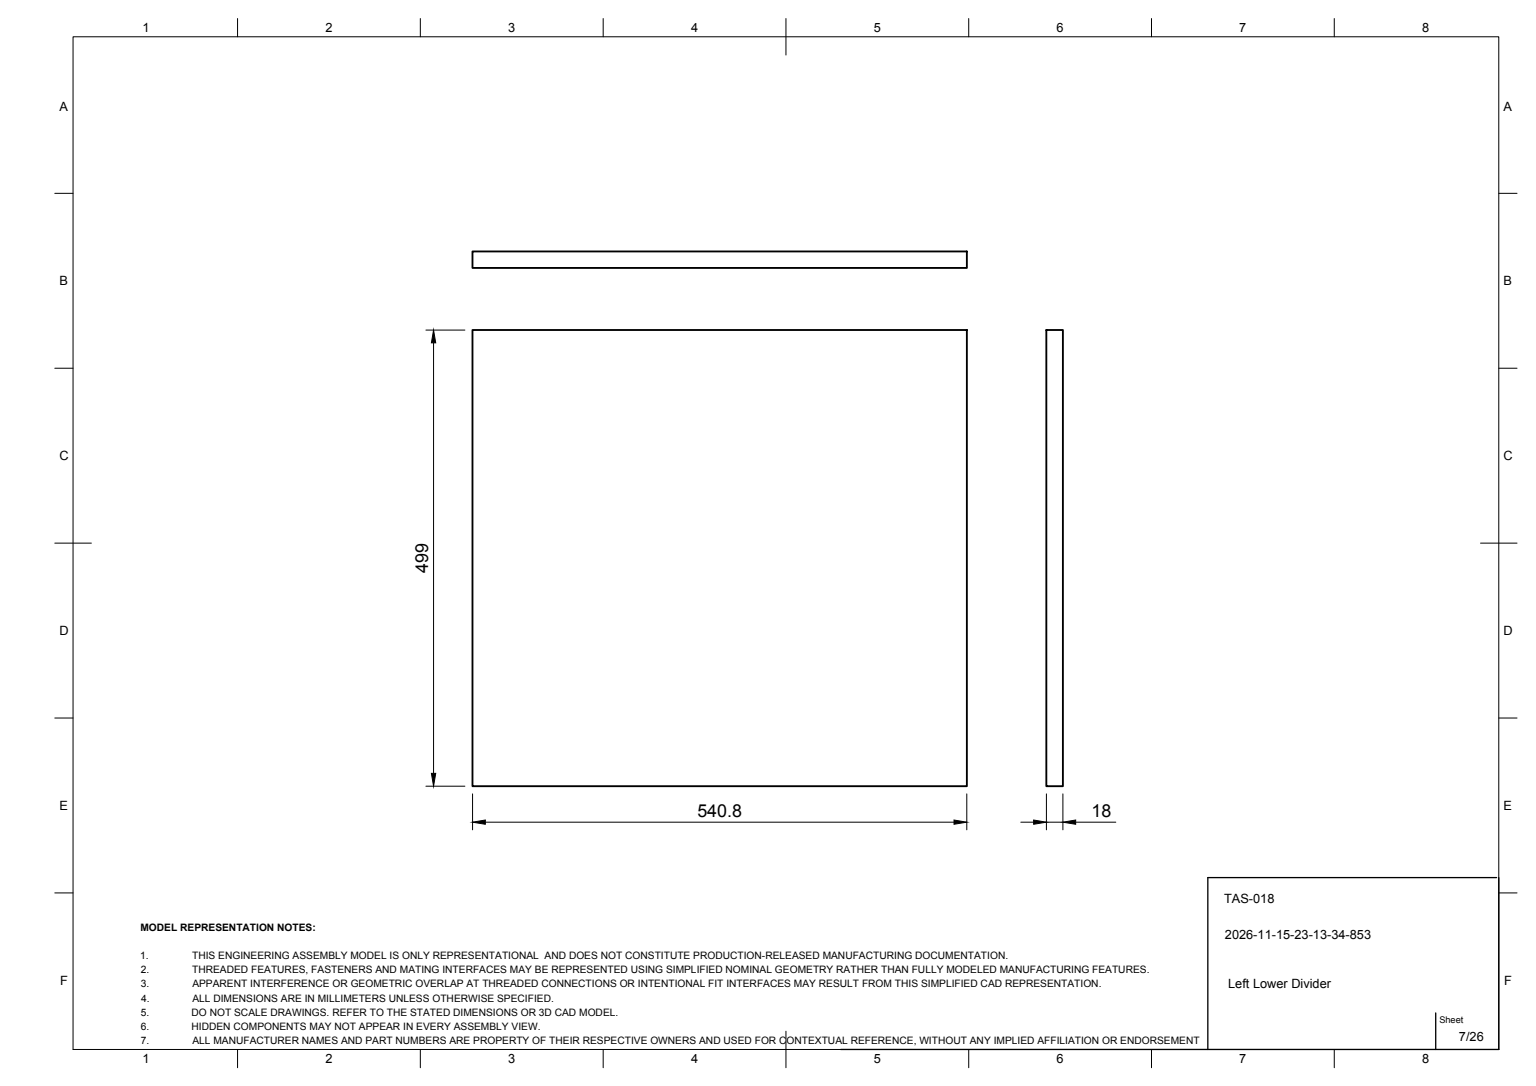
ISO-10303-21;
HEADER;
/* Generated by software containing ST-Developer
 * from STEP Tools, Inc. (www.steptools.com) 
 */

FILE_DESCRIPTION(
/* description */ (''),
/* implementation_level */ '2;1');

FILE_NAME(
/* name */ 'Left Lower Divider.step',
/* time_stamp */ '2026-11-15T15:17:57-08:00',
/* author */ (''),
/* organization */ (''),
/* preprocessor_version */ 'ST-DEVELOPER v20.2',
/* originating_system */ 'Autodesk Translation Framework v15.17.0.0',
/* authorisation */ '');

FILE_SCHEMA (('AUTOMOTIVE_DESIGN { 1 0 10303 214 3 1 1 }'));
ENDSEC;

DATA;
#10=MECHANICAL_DESIGN_GEOMETRIC_PRESENTATION_REPRESENTATION('',(#182),#3723);
#134=SHAPE_REPRESENTATION_RELATIONSHIP('SRR','None',#3815,#158);
#158=ADVANCED_BREP_SHAPE_REPRESENTATION('',(#206),#3704);
#182=STYLED_ITEM('',(#3946),#206);
#206=MANIFOLD_SOLID_BREP('Body1',#2030);
#252=FACE_OUTER_BOUND('',#378,.T.);
#253=FACE_OUTER_BOUND('',#379,.T.);
#254=FACE_OUTER_BOUND('',#380,.T.);
#255=FACE_OUTER_BOUND('',#381,.T.);
#256=FACE_OUTER_BOUND('',#382,.T.);
#257=FACE_OUTER_BOUND('',#383,.T.);
#378=EDGE_LOOP('',(#1413,#1414,#1415,#1416));
#379=EDGE_LOOP('',(#1417,#1418,#1419,#1420));
#380=EDGE_LOOP('',(#1421,#1422,#1423,#1424));
#381=EDGE_LOOP('',(#1425,#1426,#1427,#1428));
#382=EDGE_LOOP('',(#1429,#1430,#1431,#1432));
#383=EDGE_LOOP('',(#1433,#1434,#1435,#1436));
#526=LINE('',#3227,#748);
#527=LINE('',#3229,#749);
#528=LINE('',#3231,#750);
#529=LINE('',#3232,#751);
#530=LINE('',#3235,#752);
#531=LINE('',#3237,#753);
#532=LINE('',#3238,#754);
#533=LINE('',#3241,#755);
#534=LINE('',#3243,#756);
#535=LINE('',#3244,#757);
#536=LINE('',#3246,#758);
#537=LINE('',#3247,#759);
#748=VECTOR('',#2630,21.2913385826772);
#749=VECTOR('',#2631,19.6456692913386);
#750=VECTOR('',#2632,21.2913385826772);
#751=VECTOR('',#2633,19.6456692913386);
#752=VECTOR('',#2636,0.708661417322832);
#753=VECTOR('',#2637,0.708661417322832);
#754=VECTOR('',#2638,21.2913385826772);
#755=VECTOR('',#2641,19.6456692913386);
#756=VECTOR('',#2642,19.6456692913386);
#757=VECTOR('',#2643,21.2913385826772);
#758=VECTOR('',#2646,0.708661417322832);
#759=VECTOR('',#2647,0.708661417322832);
#955=VERTEX_POINT('',#3225);
#956=VERTEX_POINT('',#3226);
#957=VERTEX_POINT('',#3228);
#958=VERTEX_POINT('',#3230);
#959=VERTEX_POINT('',#3234);
#960=VERTEX_POINT('',#3236);
#961=VERTEX_POINT('',#3240);
#962=VERTEX_POINT('',#3242);
#1128=EDGE_CURVE('',#955,#956,#526,.T.);
#1129=EDGE_CURVE('',#955,#957,#527,.T.);
#1130=EDGE_CURVE('',#957,#958,#528,.T.);
#1131=EDGE_CURVE('',#956,#958,#529,.T.);
#1132=EDGE_CURVE('',#955,#959,#530,.T.);
#1133=EDGE_CURVE('',#956,#960,#531,.T.);
#1134=EDGE_CURVE('',#959,#960,#532,.T.);
#1135=EDGE_CURVE('',#959,#961,#533,.T.);
#1136=EDGE_CURVE('',#960,#962,#534,.T.);
#1137=EDGE_CURVE('',#961,#962,#535,.T.);
#1138=EDGE_CURVE('',#961,#957,#536,.T.);
#1139=EDGE_CURVE('',#962,#958,#537,.T.);
#1413=ORIENTED_EDGE('',*,*,#1128,.F.);
#1414=ORIENTED_EDGE('',*,*,#1129,.T.);
#1415=ORIENTED_EDGE('',*,*,#1130,.T.);
#1416=ORIENTED_EDGE('',*,*,#1131,.F.);
#1417=ORIENTED_EDGE('',*,*,#1132,.F.);
#1418=ORIENTED_EDGE('',*,*,#1128,.T.);
#1419=ORIENTED_EDGE('',*,*,#1133,.T.);
#1420=ORIENTED_EDGE('',*,*,#1134,.F.);
#1421=ORIENTED_EDGE('',*,*,#1135,.F.);
#1422=ORIENTED_EDGE('',*,*,#1134,.T.);
#1423=ORIENTED_EDGE('',*,*,#1136,.T.);
#1424=ORIENTED_EDGE('',*,*,#1137,.F.);
#1425=ORIENTED_EDGE('',*,*,#1138,.F.);
#1426=ORIENTED_EDGE('',*,*,#1137,.T.);
#1427=ORIENTED_EDGE('',*,*,#1139,.T.);
#1428=ORIENTED_EDGE('',*,*,#1130,.F.);
#1429=ORIENTED_EDGE('',*,*,#1131,.T.);
#1430=ORIENTED_EDGE('',*,*,#1139,.F.);
#1431=ORIENTED_EDGE('',*,*,#1136,.F.);
#1432=ORIENTED_EDGE('',*,*,#1133,.F.);
#1433=ORIENTED_EDGE('',*,*,#1129,.F.);
#1434=ORIENTED_EDGE('',*,*,#1132,.T.);
#1435=ORIENTED_EDGE('',*,*,#1135,.T.);
#1436=ORIENTED_EDGE('',*,*,#1138,.T.);
#1805=PLANE('',#2352);
#1806=PLANE('',#2353);
#1807=PLANE('',#2354);
#1808=PLANE('',#2355);
#1809=PLANE('',#2356);
#1810=PLANE('',#2357);
#1926=ADVANCED_FACE('',(#252),#1805,.T.);
#1927=ADVANCED_FACE('',(#253),#1806,.F.);
#1928=ADVANCED_FACE('',(#254),#1807,.F.);
#1929=ADVANCED_FACE('',(#255),#1808,.F.);
#1930=ADVANCED_FACE('',(#256),#1809,.F.);
#1931=ADVANCED_FACE('',(#257),#1810,.T.);
#2030=CLOSED_SHELL('',(#1926,#1927,#1928,#1929,#1930,#1931));
#2351=AXIS2_PLACEMENT_3D('',#3223,#2626,#2627);
#2352=AXIS2_PLACEMENT_3D('',#3224,#2628,#2629);
#2353=AXIS2_PLACEMENT_3D('',#3233,#2634,#2635);
#2354=AXIS2_PLACEMENT_3D('',#3239,#2639,#2640);
#2355=AXIS2_PLACEMENT_3D('',#3245,#2644,#2645);
#2356=AXIS2_PLACEMENT_3D('',#3248,#2648,#2649);
#2357=AXIS2_PLACEMENT_3D('',#3249,#2650,#2651);
#2626=DIRECTION('axis',(0.,0.,1.));
#2627=DIRECTION('refdir',(1.,0.,0.));
#2628=DIRECTION('center_axis',(-1.,0.,0.));
#2629=DIRECTION('ref_axis',(0.,0.,1.));
#2630=DIRECTION('',(0.,0.,-1.));
#2631=DIRECTION('',(0.,1.,0.));
#2632=DIRECTION('',(0.,0.,-1.));
#2633=DIRECTION('',(0.,1.,0.));
#2634=DIRECTION('center_axis',(0.,1.,0.));
#2635=DIRECTION('ref_axis',(0.,0.,1.));
#2636=DIRECTION('',(1.,0.,0.));
#2637=DIRECTION('',(1.,0.,0.));
#2638=DIRECTION('',(0.,0.,-1.));
#2639=DIRECTION('center_axis',(-1.,0.,0.));
#2640=DIRECTION('ref_axis',(0.,0.,1.));
#2641=DIRECTION('',(0.,1.,0.));
#2642=DIRECTION('',(0.,1.,0.));
#2643=DIRECTION('',(0.,0.,-1.));
#2644=DIRECTION('center_axis',(0.,-1.,0.));
#2645=DIRECTION('ref_axis',(0.,0.,-1.));
#2646=DIRECTION('',(-1.,0.,0.));
#2647=DIRECTION('',(-1.,0.,0.));
#2648=DIRECTION('center_axis',(0.,0.,1.));
#2649=DIRECTION('ref_axis',(1.,0.,0.));
#2650=DIRECTION('center_axis',(0.,0.,1.));
#2651=DIRECTION('ref_axis',(1.,0.,0.));
#3223=CARTESIAN_POINT('',(0.,0.,0.));
#3224=CARTESIAN_POINT('Origin',(-12.7086614173228,0.,46.6558556092144));
#3225=CARTESIAN_POINT('',(-12.7086614173228,4.64566929133858,22.));
#3226=CARTESIAN_POINT('',(-12.7086614173228,4.64566929133858,0.708661417322834));
#3227=CARTESIAN_POINT('',(-12.7086614173228,4.64566929133858,22.));
#3228=CARTESIAN_POINT('',(-12.7086614173228,24.2913385826772,22.));
#3229=CARTESIAN_POINT('',(-12.7086614173228,4.64566929133858,22.));
#3230=CARTESIAN_POINT('',(-12.7086614173228,24.2913385826772,0.708661417322834));
#3231=CARTESIAN_POINT('',(-12.7086614173228,24.2913385826772,22.));
#3232=CARTESIAN_POINT('',(-12.7086614173228,4.64566929133858,0.708661417322834));
#3233=CARTESIAN_POINT('Origin',(0.,4.64566929133858,46.6558556092144));
#3234=CARTESIAN_POINT('',(-12.,4.64566929133858,22.));
#3235=CARTESIAN_POINT('',(-12.7086614173228,4.64566929133858,22.));
#3236=CARTESIAN_POINT('',(-12.,4.64566929133858,0.708661417322834));
#3237=CARTESIAN_POINT('',(-12.7086614173228,4.64566929133858,0.708661417322834));
#3238=CARTESIAN_POINT('',(-12.,4.64566929133858,22.));
#3239=CARTESIAN_POINT('Origin',(-12.,0.,46.6558556092144));
#3240=CARTESIAN_POINT('',(-12.,24.2913385826772,22.));
#3241=CARTESIAN_POINT('',(-12.,4.64566929133858,22.));
#3242=CARTESIAN_POINT('',(-12.,24.2913385826772,0.708661417322834));
#3243=CARTESIAN_POINT('',(-12.,4.64566929133858,0.708661417322834));
#3244=CARTESIAN_POINT('',(-12.,24.2913385826772,22.));
#3245=CARTESIAN_POINT('Origin',(0.,24.2913385826772,46.6558556092144));
#3246=CARTESIAN_POINT('',(-12.,24.2913385826772,22.));
#3247=CARTESIAN_POINT('',(-12.,24.2913385826772,0.708661417322834));
#3248=CARTESIAN_POINT('Origin',(0.,0.,0.708661417322834));
#3249=CARTESIAN_POINT('Origin',(0.,0.,22.));
#3677=UNCERTAINTY_MEASURE_WITH_UNIT(LENGTH_MEASURE(0.000393700787401575),
#3725,'DISTANCE_ACCURACY_VALUE',
'Maximum model space distance between geometric entities at asserted c
onnectivities');
#3696=UNCERTAINTY_MEASURE_WITH_UNIT(LENGTH_MEASURE(0.000393700787401575),
#3725,'DISTANCE_ACCURACY_VALUE',
'Maximum model space distance between geometric entities at asserted c
onnectivities');
#3704=(
GEOMETRIC_REPRESENTATION_CONTEXT(3)
GLOBAL_UNCERTAINTY_ASSIGNED_CONTEXT((#3677))
GLOBAL_UNIT_ASSIGNED_CONTEXT((#3725,#3729,#3730))
REPRESENTATION_CONTEXT('','3D')
);
#3723=(
GEOMETRIC_REPRESENTATION_CONTEXT(3)
GLOBAL_UNCERTAINTY_ASSIGNED_CONTEXT((#3696))
GLOBAL_UNIT_ASSIGNED_CONTEXT((#3725,#3729,#3730))
REPRESENTATION_CONTEXT('','3D')
);
#3724=DIMENSIONAL_EXPONENTS(1.,0.,0.,0.,0.,0.,0.);
#3725=(
CONVERSION_BASED_UNIT('inch',#3728)
LENGTH_UNIT()
NAMED_UNIT(#3724)
);
#3726=(
LENGTH_UNIT()
NAMED_UNIT(*)
SI_UNIT(.MILLI.,.METRE.)
);
#3728=LENGTH_MEASURE_WITH_UNIT(LENGTH_MEASURE(25.4),#3726);
#3729=(
NAMED_UNIT(*)
PLANE_ANGLE_UNIT()
SI_UNIT($,.RADIAN.)
);
#3730=(
NAMED_UNIT(*)
SI_UNIT($,.STERADIAN.)
SOLID_ANGLE_UNIT()
);
#3738=SHAPE_DEFINITION_REPRESENTATION(#3765,#3815);
#3765=PRODUCT_DEFINITION_SHAPE('',$,#3842);
#3815=SHAPE_REPRESENTATION('',(#2351),#3704);
#3834=PRODUCT_DEFINITION_CONTEXT('part definition',#3914,'design');
#3842=PRODUCT_DEFINITION('2026-11-15-23-13-34-853','Left Lower Divider',
#3868,#3834);
#3868=PRODUCT_DEFINITION_FORMATION('',$,#3923);
#3914=APPLICATION_CONTEXT(
'Core Data for Automotive Mechanical Design Process');
#3915=PRODUCT_CONTEXT('part definition',#3914,'mechanical');
#3923=PRODUCT('2026-11-15-23-13-34-853','Left Lower Divider',$,(#3915));
#3946=PRESENTATION_STYLE_ASSIGNMENT((#3954));
#3954=SURFACE_STYLE_USAGE(.BOTH.,#3962);
#3962=SURFACE_SIDE_STYLE('',(#3970));
#3970=SURFACE_STYLE_FILL_AREA(#3978);
#3978=FILL_AREA_STYLE('Gray',(#3986));
#3986=FILL_AREA_STYLE_COLOUR('Gray',#3994);
#3994=COLOUR_RGB('Gray',0.501960784313725,0.501960784313725,0.501960784313725);
ENDSEC;
END-ISO-10303-21;
